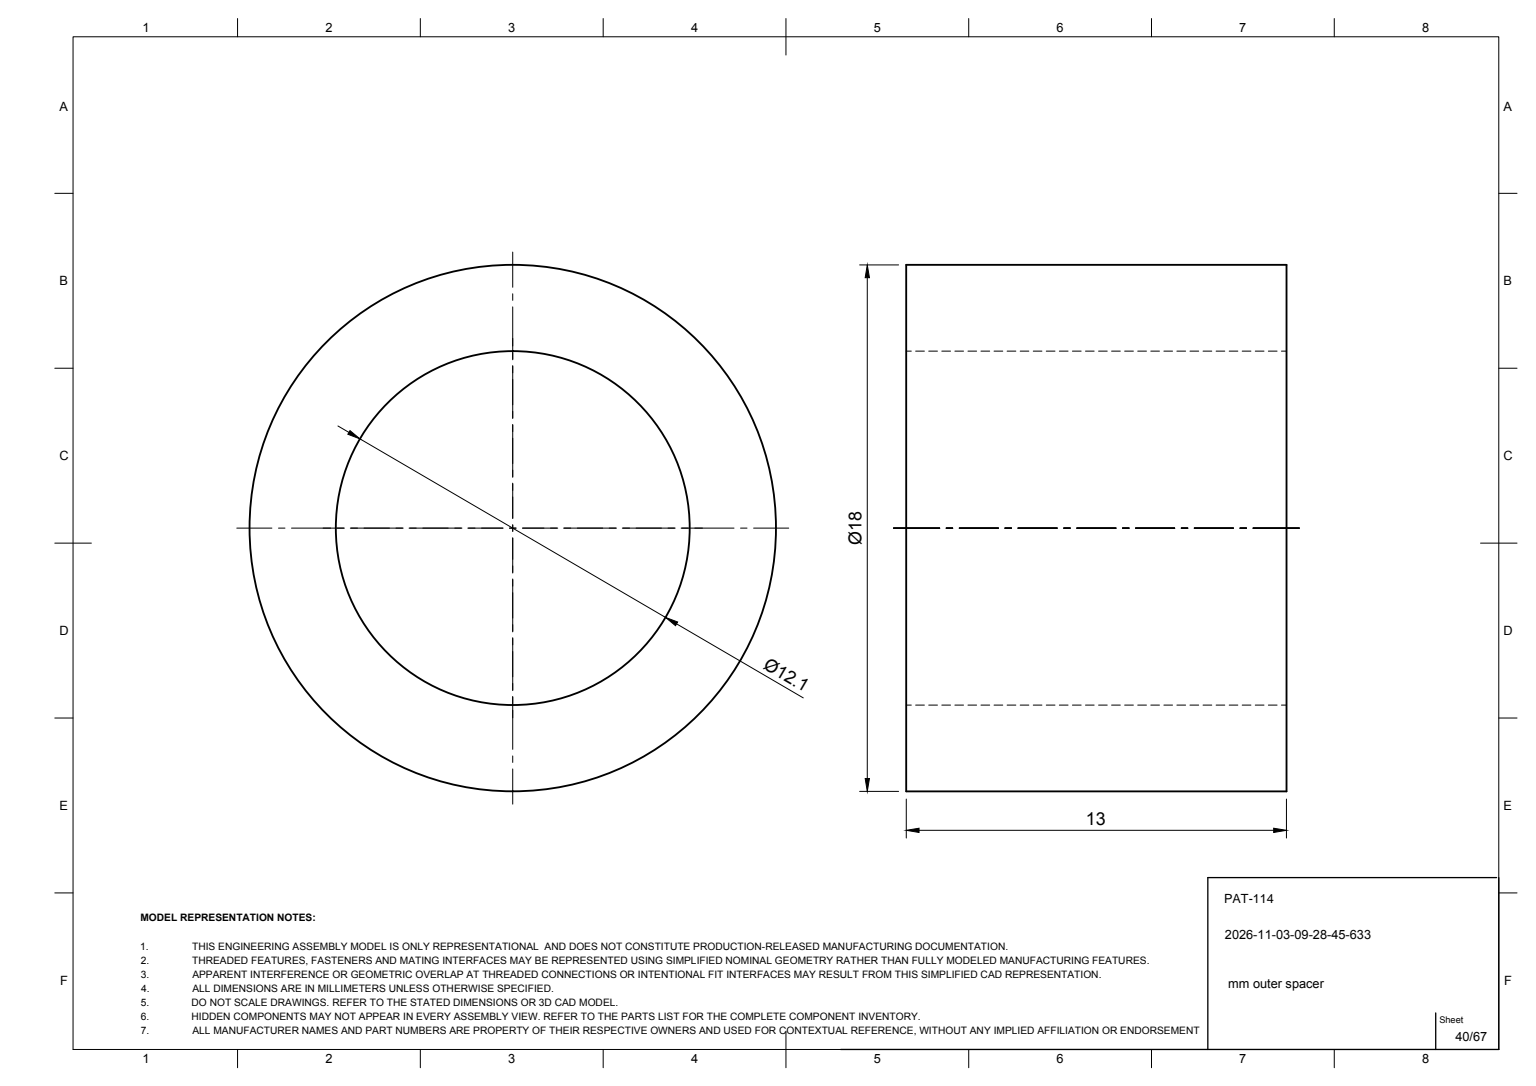
ISO-10303-21;
HEADER;
/* Generated by software containing ST-Developer
 * from STEP Tools, Inc. (www.steptools.com) 
 */

FILE_DESCRIPTION(
/* description */ ('Two-stage gear reducer in split housing'),
/* implementation_level */ '2;1');

FILE_NAME(
/* name */ 'mm outer spacer.step',
/* time_stamp */ '2026-10-28T03:22:31-07:00',
/* author */ (''),
/* organization */ (''),
/* preprocessor_version */ 'ST-DEVELOPER v20.2',
/* originating_system */ 'Autodesk Translation Framework v15.17.0.0',
/* authorisation */ '');

FILE_SCHEMA (('AUTOMOTIVE_DESIGN { 1 0 10303 214 3 1 1 }'));
ENDSEC;

DATA;
#10=MECHANICAL_DESIGN_GEOMETRIC_PRESENTATION_REPRESENTATION('',(#1280),#73366);
#1153=SHAPE_REPRESENTATION_RELATIONSHIP('SRR','None',#73643,#1209);
#1209=ADVANCED_BREP_SHAPE_REPRESENTATION('',(#1349),#73339);
#1280=STYLED_ITEM('',(#73974),#1349);
#1349=MANIFOLD_SOLID_BREP('Body1',#16170);
#1547=FACE_BOUND('',#3527,.T.);
#1548=FACE_BOUND('',#3529,.T.);
#1814=PLANE('',#17815);
#1815=PLANE('',#17816);
#2438=FACE_OUTER_BOUND('',#3524,.T.);
#2439=FACE_OUTER_BOUND('',#3525,.T.);
#2440=FACE_OUTER_BOUND('',#3526,.T.);
#2441=FACE_OUTER_BOUND('',#3528,.T.);
#3524=EDGE_LOOP('',(#12383,#12384,#12385,#12386));
#3525=EDGE_LOOP('',(#12387,#12388,#12389,#12390));
#3526=EDGE_LOOP('',(#12391));
#3527=EDGE_LOOP('',(#12392));
#3528=EDGE_LOOP('',(#12393));
#3529=EDGE_LOOP('',(#12394));
#4500=LINE('',#25636,#5524);
#4501=LINE('',#25642,#5525);
#5524=VECTOR('',#20900,0.605);
#5525=VECTOR('',#20907,0.9);
#6558=CIRCLE('',#17810,0.605);
#6559=CIRCLE('',#17811,0.605);
#6560=CIRCLE('',#17813,0.9);
#6561=CIRCLE('',#17814,0.9);
#7465=VERTEX_POINT('',#25633);
#7466=VERTEX_POINT('',#25635);
#7467=VERTEX_POINT('',#25639);
#7468=VERTEX_POINT('',#25641);
#9245=EDGE_CURVE('',#7465,#7465,#6558,.T.);
#9246=EDGE_CURVE('',#7465,#7466,#4500,.T.);
#9247=EDGE_CURVE('',#7466,#7466,#6559,.T.);
#9248=EDGE_CURVE('',#7467,#7467,#6560,.T.);
#9249=EDGE_CURVE('',#7467,#7468,#4501,.T.);
#9250=EDGE_CURVE('',#7468,#7468,#6561,.T.);
#12383=ORIENTED_EDGE('',*,*,#9245,.F.);
#12384=ORIENTED_EDGE('',*,*,#9246,.T.);
#12385=ORIENTED_EDGE('',*,*,#9247,.T.);
#12386=ORIENTED_EDGE('',*,*,#9246,.F.);
#12387=ORIENTED_EDGE('',*,*,#9248,.F.);
#12388=ORIENTED_EDGE('',*,*,#9249,.T.);
#12389=ORIENTED_EDGE('',*,*,#9250,.T.);
#12390=ORIENTED_EDGE('',*,*,#9249,.F.);
#12391=ORIENTED_EDGE('',*,*,#9248,.T.);
#12392=ORIENTED_EDGE('',*,*,#9245,.T.);
#12393=ORIENTED_EDGE('',*,*,#9250,.F.);
#12394=ORIENTED_EDGE('',*,*,#9247,.F.);
#15082=CYLINDRICAL_SURFACE('',#17809,0.605);
#15083=CYLINDRICAL_SURFACE('',#17812,0.9);
#15645=ADVANCED_FACE('',(#2438),#15082,.F.);
#15646=ADVANCED_FACE('',(#2439),#15083,.T.);
#15647=ADVANCED_FACE('',(#2440,#1547),#1814,.T.);
#15648=ADVANCED_FACE('',(#2441,#1548),#1815,.F.);
#16170=CLOSED_SHELL('',(#15645,#15646,#15647,#15648));
#17808=AXIS2_PLACEMENT_3D('',#25631,#20894,#20895);
#17809=AXIS2_PLACEMENT_3D('',#25632,#20896,#20897);
#17810=AXIS2_PLACEMENT_3D('',#25634,#20898,#20899);
#17811=AXIS2_PLACEMENT_3D('',#25637,#20901,#20902);
#17812=AXIS2_PLACEMENT_3D('',#25638,#20903,#20904);
#17813=AXIS2_PLACEMENT_3D('',#25640,#20905,#20906);
#17814=AXIS2_PLACEMENT_3D('',#25643,#20908,#20909);
#17815=AXIS2_PLACEMENT_3D('',#25644,#20910,#20911);
#17816=AXIS2_PLACEMENT_3D('',#25645,#20912,#20913);
#20894=DIRECTION('axis',(0.,0.,1.));
#20895=DIRECTION('refdir',(1.,0.,0.));
#20896=DIRECTION('center_axis',(0.,1.,0.));
#20897=DIRECTION('ref_axis',(1.,0.,0.));
#20898=DIRECTION('center_axis',(0.,-1.,0.));
#20899=DIRECTION('ref_axis',(1.,0.,0.));
#20900=DIRECTION('',(0.,-1.,0.));
#20901=DIRECTION('center_axis',(0.,-1.,0.));
#20902=DIRECTION('ref_axis',(1.,0.,0.));
#20903=DIRECTION('center_axis',(0.,1.,0.));
#20904=DIRECTION('ref_axis',(1.,0.,0.));
#20905=DIRECTION('center_axis',(0.,1.,0.));
#20906=DIRECTION('ref_axis',(1.,0.,0.));
#20907=DIRECTION('',(0.,-1.,0.));
#20908=DIRECTION('center_axis',(0.,1.,0.));
#20909=DIRECTION('ref_axis',(1.,0.,0.));
#20910=DIRECTION('center_axis',(0.,1.,0.));
#20911=DIRECTION('ref_axis',(1.,0.,0.));
#20912=DIRECTION('center_axis',(0.,1.,0.));
#20913=DIRECTION('ref_axis',(1.,0.,0.));
#25631=CARTESIAN_POINT('',(0.,0.,0.));
#25632=CARTESIAN_POINT('Origin',(0.,-7.8,10.));
#25633=CARTESIAN_POINT('',(-0.605,-6.5,10.));
#25634=CARTESIAN_POINT('Origin',(0.,-6.5,10.));
#25635=CARTESIAN_POINT('',(-0.605,-7.8,10.));
#25636=CARTESIAN_POINT('',(-0.605,-7.8,10.));
#25637=CARTESIAN_POINT('Origin',(0.,-7.8,10.));
#25638=CARTESIAN_POINT('Origin',(0.,-7.8,10.));
#25639=CARTESIAN_POINT('',(-0.9,-6.5,10.));
#25640=CARTESIAN_POINT('Origin',(0.,-6.5,10.));
#25641=CARTESIAN_POINT('',(-0.9,-7.8,10.));
#25642=CARTESIAN_POINT('',(-0.9,-7.8,10.));
#25643=CARTESIAN_POINT('Origin',(0.,-7.8,10.));
#25644=CARTESIAN_POINT('Origin',(0.,-6.5,10.));
#25645=CARTESIAN_POINT('Origin',(0.,-7.8,10.));
#73275=UNCERTAINTY_MEASURE_WITH_UNIT(LENGTH_MEASURE(0.001),#73367,
'DISTANCE_ACCURACY_VALUE',
'Maximum model space distance between geometric entities at asserted c
onnectivities');
#73302=UNCERTAINTY_MEASURE_WITH_UNIT(LENGTH_MEASURE(0.001),#73367,
'DISTANCE_ACCURACY_VALUE',
'Maximum model space distance between geometric entities at asserted c
onnectivities');
#73339=(
GEOMETRIC_REPRESENTATION_CONTEXT(3)
GLOBAL_UNCERTAINTY_ASSIGNED_CONTEXT((#73275))
GLOBAL_UNIT_ASSIGNED_CONTEXT((#73367,#73369,#73370))
REPRESENTATION_CONTEXT('','3D')
);
#73366=(
GEOMETRIC_REPRESENTATION_CONTEXT(3)
GLOBAL_UNCERTAINTY_ASSIGNED_CONTEXT((#73302))
GLOBAL_UNIT_ASSIGNED_CONTEXT((#73367,#73369,#73370))
REPRESENTATION_CONTEXT('','3D')
);
#73367=(
LENGTH_UNIT()
NAMED_UNIT(*)
SI_UNIT(.CENTI.,.METRE.)
);
#73369=(
NAMED_UNIT(*)
PLANE_ANGLE_UNIT()
SI_UNIT($,.RADIAN.)
);
#73370=(
NAMED_UNIT(*)
SI_UNIT($,.STERADIAN.)
SOLID_ANGLE_UNIT()
);
#73407=SHAPE_DEFINITION_REPRESENTATION(#73540,#73643);
#73540=PRODUCT_DEFINITION_SHAPE('',$,#73707);
#73643=SHAPE_REPRESENTATION('',(#17808),#73339);
#73670=PRODUCT_DEFINITION_CONTEXT('part definition',#73861,'design');
#73707=PRODUCT_DEFINITION('mm outer spacer','mm outer spacer',#73770,#73670);
#73770=PRODUCT_DEFINITION_FORMATION('',$,#73899);
#73861=APPLICATION_CONTEXT(
'Core Data for Automotive Mechanical Design Process');
#73862=PRODUCT_CONTEXT('part definition',#73861,'mechanical');
#73899=PRODUCT('mm outer spacer','mm outer spacer','mm outer spacer',(#73862));
#73968=COLOUR_RGB('Light Blue',0.38,0.62,0.78);
#73969=FILL_AREA_STYLE_COLOUR('',#73968);
#73970=FILL_AREA_STYLE('',(#73969));
#73971=SURFACE_STYLE_FILL_AREA(#73970);
#73972=SURFACE_SIDE_STYLE('',(#73971));
#73973=SURFACE_STYLE_USAGE(.BOTH.,#73972);
#73974=PRESENTATION_STYLE_ASSIGNMENT((#73973));
ENDSEC;
END-ISO-10303-21;
